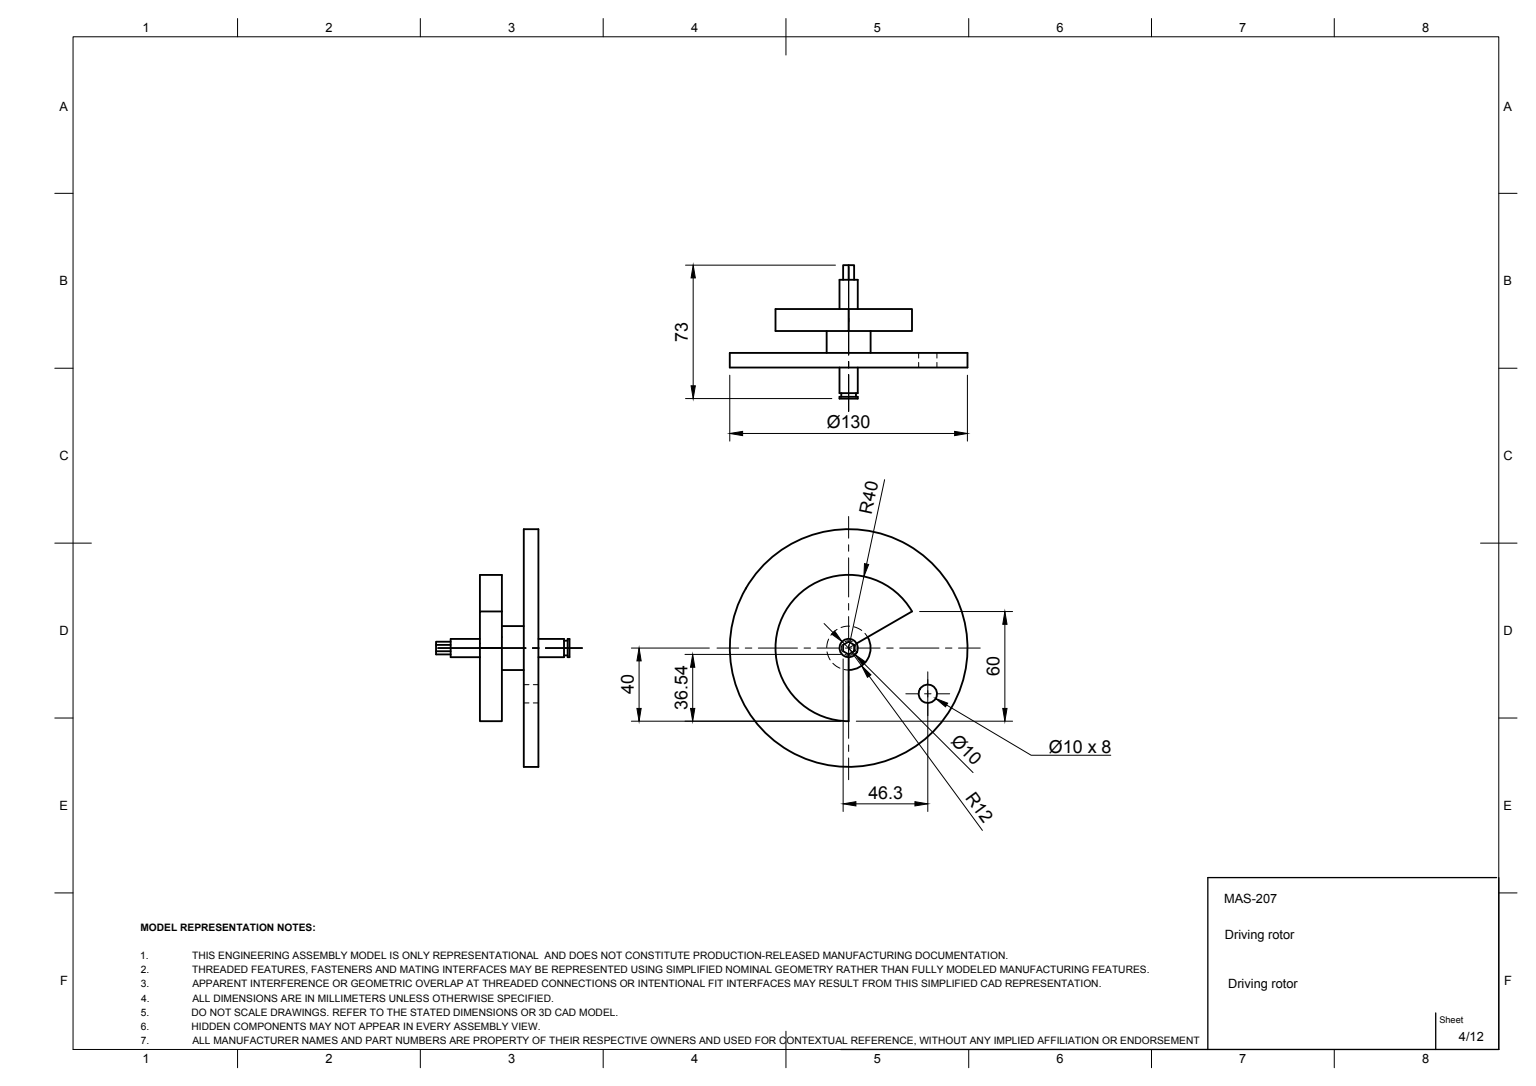
ISO-10303-21;
HEADER;
/* Generated by software containing ST-Developer
 * from STEP Tools, Inc. (www.steptools.com) 
 */

FILE_DESCRIPTION(
/* description */ ('Independent six-slot Geneva indexer. Center distance100, drive radius
50, 60degree indexing per input revolution with120degree engagement an
d240degree dwell. Native machined concave locking faces and relieved d
isk; replaceable retained drive pin; keyed output shaft. Geometry traj
ectory checks use calculated indexing positions, not a contact-dynamic
s simulation. No load or production rating assigned.'),
/* implementation_level */ '2;1');

FILE_NAME(
/* name */ 'Driving rotor.step',
/* time_stamp */ '2026-11-09T17:53:22-08:00',
/* author */ (''),
/* organization */ (''),
/* preprocessor_version */ 'ST-DEVELOPER v20.2',
/* originating_system */ 'Autodesk Translation Framework v15.17.0.0',
/* authorisation */ '');

FILE_SCHEMA (('AUTOMOTIVE_DESIGN { 1 0 10303 214 3 1 1 }'));
ENDSEC;

DATA;
#10=MECHANICAL_DESIGN_GEOMETRIC_PRESENTATION_REPRESENTATION('',(#102),#4149);
#80=SHAPE_REPRESENTATION_RELATIONSHIP('SRR','None',#4197,#91);
#91=ADVANCED_BREP_SHAPE_REPRESENTATION('',(#113),#4139);
#102=STYLED_ITEM('',(#4261),#113);
#113=MANIFOLD_SOLID_BREP('Body1',#2296);
#135=FACE_BOUND('',#407,.T.);
#136=FACE_BOUND('',#409,.T.);
#137=FACE_BOUND('',#421,.T.);
#138=FACE_BOUND('',#422,.T.);
#139=FACE_BOUND('',#424,.T.);
#140=FACE_BOUND('',#425,.T.);
#141=FACE_BOUND('',#430,.T.);
#167=PLANE('',#2455);
#168=PLANE('',#2456);
#169=PLANE('',#2457);
#170=PLANE('',#2458);
#171=PLANE('',#2459);
#172=PLANE('',#2460);
#173=PLANE('',#2461);
#174=PLANE('',#2465);
#175=PLANE('',#2467);
#176=PLANE('',#2474);
#177=PLANE('',#2476);
#178=PLANE('',#2478);
#179=PLANE('',#2479);
#180=PLANE('',#2480);
#181=PLANE('',#2484);
#182=PLANE('',#2491);
#183=PLANE('',#2493);
#184=PLANE('',#2500);
#185=PLANE('',#2501);
#250=FACE_OUTER_BOUND('',#398,.T.);
#251=FACE_OUTER_BOUND('',#399,.T.);
#252=FACE_OUTER_BOUND('',#400,.T.);
#253=FACE_OUTER_BOUND('',#401,.T.);
#254=FACE_OUTER_BOUND('',#402,.T.);
#255=FACE_OUTER_BOUND('',#403,.T.);
#256=FACE_OUTER_BOUND('',#404,.T.);
#257=FACE_OUTER_BOUND('',#405,.T.);
#258=FACE_OUTER_BOUND('',#406,.T.);
#259=FACE_OUTER_BOUND('',#408,.T.);
#260=FACE_OUTER_BOUND('',#410,.T.);
#261=FACE_OUTER_BOUND('',#411,.T.);
#262=FACE_OUTER_BOUND('',#412,.T.);
#263=FACE_OUTER_BOUND('',#413,.T.);
#264=FACE_OUTER_BOUND('',#414,.T.);
#265=FACE_OUTER_BOUND('',#415,.T.);
#266=FACE_OUTER_BOUND('',#416,.T.);
#267=FACE_OUTER_BOUND('',#417,.T.);
#268=FACE_OUTER_BOUND('',#418,.T.);
#269=FACE_OUTER_BOUND('',#419,.T.);
#270=FACE_OUTER_BOUND('',#420,.T.);
#271=FACE_OUTER_BOUND('',#423,.T.);
#272=FACE_OUTER_BOUND('',#426,.T.);
#273=FACE_OUTER_BOUND('',#427,.T.);
#274=FACE_OUTER_BOUND('',#428,.T.);
#275=FACE_OUTER_BOUND('',#429,.T.);
#276=FACE_OUTER_BOUND('',#431,.T.);
#398=EDGE_LOOP('',(#1568,#1569,#1570,#1571));
#399=EDGE_LOOP('',(#1572,#1573,#1574,#1575));
#400=EDGE_LOOP('',(#1576,#1577,#1578,#1579));
#401=EDGE_LOOP('',(#1580,#1581,#1582,#1583));
#402=EDGE_LOOP('',(#1584,#1585,#1586,#1587));
#403=EDGE_LOOP('',(#1588,#1589,#1590,#1591));
#404=EDGE_LOOP('',(#1592,#1593,#1594,#1595,#1596,#1597));
#405=EDGE_LOOP('',(#1598,#1599,#1600,#1601));
#406=EDGE_LOOP('',(#1602));
#407=EDGE_LOOP('',(#1603));
#408=EDGE_LOOP('',(#1604));
#409=EDGE_LOOP('',(#1605));
#410=EDGE_LOOP('',(#1606,#1607,#1608,#1609));
#411=EDGE_LOOP('',(#1610,#1611,#1612,#1613));
#412=EDGE_LOOP('',(#1614,#1615,#1616));
#413=EDGE_LOOP('',(#1617,#1618,#1619));
#414=EDGE_LOOP('',(#1620,#1621,#1622,#1623,#1624,#1625));
#415=EDGE_LOOP('',(#1626,#1627,#1628,#1629,#1630,#1631));
#416=EDGE_LOOP('',(#1632,#1633,#1634,#1635,#1636));
#417=EDGE_LOOP('',(#1637,#1638,#1639,#1640,#1641));
#418=EDGE_LOOP('',(#1642,#1643,#1644,#1645));
#419=EDGE_LOOP('',(#1646,#1647,#1648,#1649,#1650,#1651));
#420=EDGE_LOOP('',(#1652));
#421=EDGE_LOOP('',(#1653));
#422=EDGE_LOOP('',(#1654));
#423=EDGE_LOOP('',(#1655));
#424=EDGE_LOOP('',(#1656));
#425=EDGE_LOOP('',(#1657));
#426=EDGE_LOOP('',(#1658,#1659,#1660,#1661));
#427=EDGE_LOOP('',(#1662,#1663,#1664,#1665));
#428=EDGE_LOOP('',(#1666,#1667,#1668,#1669,#1670,#1671));
#429=EDGE_LOOP('',(#1672));
#430=EDGE_LOOP('',(#1673,#1674,#1675,#1676,#1677,#1678));
#431=EDGE_LOOP('',(#1679));
#566=LINE('',#3535,#738);
#567=LINE('',#3537,#739);
#568=LINE('',#3539,#740);
#569=LINE('',#3540,#741);
#570=LINE('',#3543,#742);
#571=LINE('',#3545,#743);
#572=LINE('',#3546,#744);
#573=LINE('',#3549,#745);
#574=LINE('',#3551,#746);
#575=LINE('',#3552,#747);
#576=LINE('',#3555,#748);
#577=LINE('',#3557,#749);
#578=LINE('',#3558,#750);
#579=LINE('',#3561,#751);
#580=LINE('',#3563,#752);
#581=LINE('',#3564,#753);
#582=LINE('',#3566,#754);
#583=LINE('',#3567,#755);
#584=LINE('',#3573,#756);
#585=LINE('',#3584,#757);
#586=LINE('',#3589,#758);
#587=LINE('',#3596,#759);
#588=LINE('',#3597,#760);
#589=LINE('',#3603,#761);
#590=LINE('',#3604,#762);
#591=LINE('',#3608,#763);
#592=LINE('',#3609,#764);
#593=LINE('',#3610,#765);
#594=LINE('',#3611,#766);
#595=LINE('',#3615,#767);
#596=LINE('',#3616,#768);
#597=LINE('',#3617,#769);
#598=LINE('',#3631,#770);
#599=LINE('',#3640,#771);
#600=LINE('',#3643,#772);
#601=LINE('',#3648,#773);
#738=VECTOR('',#2791,10.);
#739=VECTOR('',#2792,10.);
#740=VECTOR('',#2793,10.);
#741=VECTOR('',#2794,10.);
#742=VECTOR('',#2797,10.);
#743=VECTOR('',#2798,10.);
#744=VECTOR('',#2799,10.);
#745=VECTOR('',#2802,10.);
#746=VECTOR('',#2803,10.);
#747=VECTOR('',#2804,10.);
#748=VECTOR('',#2807,10.);
#749=VECTOR('',#2808,10.);
#750=VECTOR('',#2809,10.);
#751=VECTOR('',#2812,10.);
#752=VECTOR('',#2813,10.);
#753=VECTOR('',#2814,10.);
#754=VECTOR('',#2817,10.);
#755=VECTOR('',#2818,10.);
#756=VECTOR('',#2825,4.);
#757=VECTOR('',#2840,5.);
#758=VECTOR('',#2845,5.);
#759=VECTOR('',#2852,10.);
#760=VECTOR('',#2853,10.);
#761=VECTOR('',#2858,10.);
#762=VECTOR('',#2859,10.);
#763=VECTOR('',#2862,10.);
#764=VECTOR('',#2863,10.);
#765=VECTOR('',#2864,10.);
#766=VECTOR('',#2865,10.);
#767=VECTOR('',#2868,10.);
#768=VECTOR('',#2869,10.);
#769=VECTOR('',#2870,10.);
#770=VECTOR('',#2891,12.);
#771=VECTOR('',#2904,60.);
#772=VECTOR('',#2907,5.);
#773=VECTOR('',#2914,5.);
#904=CIRCLE('',#2463,4.);
#905=CIRCLE('',#2464,4.);
#906=CIRCLE('',#2466,5.);
#907=CIRCLE('',#2468,5.);
#908=CIRCLE('',#2470,5.);
#909=CIRCLE('',#2472,5.);
#910=CIRCLE('',#2473,5.);
#911=CIRCLE('',#2475,5.);
#912=CIRCLE('',#2477,12.);
#913=CIRCLE('',#2481,5.);
#914=CIRCLE('',#2482,5.);
#915=CIRCLE('',#2483,40.);
#916=CIRCLE('',#2485,40.);
#917=CIRCLE('',#2486,12.);
#918=CIRCLE('',#2487,12.);
#919=CIRCLE('',#2490,12.);
#920=CIRCLE('',#2492,65.);
#921=CIRCLE('',#2494,65.);
#922=CIRCLE('',#2497,5.);
#923=CIRCLE('',#2499,5.);
#1036=VERTEX_POINT('',#3533);
#1037=VERTEX_POINT('',#3534);
#1038=VERTEX_POINT('',#3536);
#1039=VERTEX_POINT('',#3538);
#1040=VERTEX_POINT('',#3542);
#1041=VERTEX_POINT('',#3544);
#1042=VERTEX_POINT('',#3548);
#1043=VERTEX_POINT('',#3550);
#1044=VERTEX_POINT('',#3554);
#1045=VERTEX_POINT('',#3556);
#1046=VERTEX_POINT('',#3560);
#1047=VERTEX_POINT('',#3562);
#1048=VERTEX_POINT('',#3570);
#1049=VERTEX_POINT('',#3572);
#1050=VERTEX_POINT('',#3576);
#1051=VERTEX_POINT('',#3579);
#1052=VERTEX_POINT('',#3582);
#1053=VERTEX_POINT('',#3586);
#1054=VERTEX_POINT('',#3588);
#1055=VERTEX_POINT('',#3592);
#1056=VERTEX_POINT('',#3593);
#1057=VERTEX_POINT('',#3595);
#1058=VERTEX_POINT('',#3599);
#1059=VERTEX_POINT('',#3600);
#1060=VERTEX_POINT('',#3602);
#1061=VERTEX_POINT('',#3606);
#1062=VERTEX_POINT('',#3607);
#1063=VERTEX_POINT('',#3613);
#1064=VERTEX_POINT('',#3614);
#1065=VERTEX_POINT('',#3619);
#1066=VERTEX_POINT('',#3625);
#1067=VERTEX_POINT('',#3630);
#1068=VERTEX_POINT('',#3634);
#1069=VERTEX_POINT('',#3637);
#1070=VERTEX_POINT('',#3642);
#1071=VERTEX_POINT('',#3646);
#1242=EDGE_CURVE('',#1036,#1037,#566,.T.);
#1243=EDGE_CURVE('',#1036,#1038,#567,.T.);
#1244=EDGE_CURVE('',#1039,#1038,#568,.T.);
#1245=EDGE_CURVE('',#1037,#1039,#569,.T.);
#1246=EDGE_CURVE('',#1037,#1040,#570,.T.);
#1247=EDGE_CURVE('',#1041,#1039,#571,.T.);
#1248=EDGE_CURVE('',#1040,#1041,#572,.T.);
#1249=EDGE_CURVE('',#1040,#1042,#573,.T.);
#1250=EDGE_CURVE('',#1043,#1041,#574,.T.);
#1251=EDGE_CURVE('',#1042,#1043,#575,.T.);
#1252=EDGE_CURVE('',#1042,#1044,#576,.T.);
#1253=EDGE_CURVE('',#1045,#1043,#577,.T.);
#1254=EDGE_CURVE('',#1044,#1045,#578,.T.);
#1255=EDGE_CURVE('',#1044,#1046,#579,.T.);
#1256=EDGE_CURVE('',#1047,#1045,#580,.T.);
#1257=EDGE_CURVE('',#1046,#1047,#581,.T.);
#1258=EDGE_CURVE('',#1046,#1036,#582,.T.);
#1259=EDGE_CURVE('',#1038,#1047,#583,.T.);
#1260=EDGE_CURVE('',#1048,#1048,#904,.T.);
#1261=EDGE_CURVE('',#1048,#1049,#584,.T.);
#1262=EDGE_CURVE('',#1049,#1049,#905,.T.);
#1263=EDGE_CURVE('',#1050,#1050,#906,.T.);
#1264=EDGE_CURVE('',#1051,#1051,#907,.T.);
#1265=EDGE_CURVE('',#1052,#1052,#908,.T.);
#1266=EDGE_CURVE('',#1052,#1051,#585,.T.);
#1267=EDGE_CURVE('',#1053,#1053,#909,.T.);
#1268=EDGE_CURVE('',#1053,#1054,#586,.T.);
#1269=EDGE_CURVE('',#1054,#1054,#910,.T.);
#1270=EDGE_CURVE('',#1055,#1056,#911,.T.);
#1271=EDGE_CURVE('',#1057,#1055,#587,.T.);
#1272=EDGE_CURVE('',#1056,#1057,#588,.T.);
#1273=EDGE_CURVE('',#1058,#1059,#912,.T.);
#1274=EDGE_CURVE('',#1060,#1059,#589,.T.);
#1275=EDGE_CURVE('',#1058,#1060,#590,.T.);
#1276=EDGE_CURVE('',#1061,#1062,#591,.T.);
#1277=EDGE_CURVE('',#1056,#1061,#592,.T.);
#1278=EDGE_CURVE('',#1057,#1060,#593,.T.);
#1279=EDGE_CURVE('',#1062,#1059,#594,.T.);
#1280=EDGE_CURVE('',#1063,#1064,#595,.T.);
#1281=EDGE_CURVE('',#1058,#1063,#596,.T.);
#1282=EDGE_CURVE('',#1064,#1055,#597,.T.);
#1283=EDGE_CURVE('',#1065,#1055,#913,.T.);
#1284=EDGE_CURVE('',#1056,#1065,#914,.T.);
#1285=EDGE_CURVE('',#1061,#1064,#915,.T.);
#1286=EDGE_CURVE('',#1062,#1063,#916,.T.);
#1287=EDGE_CURVE('',#1059,#1066,#917,.T.);
#1288=EDGE_CURVE('',#1066,#1058,#918,.T.);
#1289=EDGE_CURVE('',#1066,#1067,#598,.T.);
#1290=EDGE_CURVE('',#1067,#1067,#919,.T.);
#1291=EDGE_CURVE('',#1068,#1068,#920,.F.);
#1292=EDGE_CURVE('',#1069,#1069,#921,.F.);
#1293=EDGE_CURVE('',#1068,#1069,#599,.T.);
#1294=EDGE_CURVE('',#1050,#1070,#600,.T.);
#1295=EDGE_CURVE('',#1070,#1070,#922,.T.);
#1296=EDGE_CURVE('',#1071,#1071,#923,.T.);
#1297=EDGE_CURVE('',#1071,#1065,#601,.T.);
#1568=ORIENTED_EDGE('',*,*,#1242,.F.);
#1569=ORIENTED_EDGE('',*,*,#1243,.T.);
#1570=ORIENTED_EDGE('',*,*,#1244,.F.);
#1571=ORIENTED_EDGE('',*,*,#1245,.F.);
#1572=ORIENTED_EDGE('',*,*,#1246,.F.);
#1573=ORIENTED_EDGE('',*,*,#1245,.T.);
#1574=ORIENTED_EDGE('',*,*,#1247,.F.);
#1575=ORIENTED_EDGE('',*,*,#1248,.F.);
#1576=ORIENTED_EDGE('',*,*,#1249,.F.);
#1577=ORIENTED_EDGE('',*,*,#1248,.T.);
#1578=ORIENTED_EDGE('',*,*,#1250,.F.);
#1579=ORIENTED_EDGE('',*,*,#1251,.F.);
#1580=ORIENTED_EDGE('',*,*,#1252,.F.);
#1581=ORIENTED_EDGE('',*,*,#1251,.T.);
#1582=ORIENTED_EDGE('',*,*,#1253,.F.);
#1583=ORIENTED_EDGE('',*,*,#1254,.F.);
#1584=ORIENTED_EDGE('',*,*,#1255,.F.);
#1585=ORIENTED_EDGE('',*,*,#1254,.T.);
#1586=ORIENTED_EDGE('',*,*,#1256,.F.);
#1587=ORIENTED_EDGE('',*,*,#1257,.F.);
#1588=ORIENTED_EDGE('',*,*,#1258,.F.);
#1589=ORIENTED_EDGE('',*,*,#1257,.T.);
#1590=ORIENTED_EDGE('',*,*,#1259,.F.);
#1591=ORIENTED_EDGE('',*,*,#1243,.F.);
#1592=ORIENTED_EDGE('',*,*,#1259,.T.);
#1593=ORIENTED_EDGE('',*,*,#1256,.T.);
#1594=ORIENTED_EDGE('',*,*,#1253,.T.);
#1595=ORIENTED_EDGE('',*,*,#1250,.T.);
#1596=ORIENTED_EDGE('',*,*,#1247,.T.);
#1597=ORIENTED_EDGE('',*,*,#1244,.T.);
#1598=ORIENTED_EDGE('',*,*,#1260,.T.);
#1599=ORIENTED_EDGE('',*,*,#1261,.T.);
#1600=ORIENTED_EDGE('',*,*,#1262,.F.);
#1601=ORIENTED_EDGE('',*,*,#1261,.F.);
#1602=ORIENTED_EDGE('',*,*,#1263,.F.);
#1603=ORIENTED_EDGE('',*,*,#1260,.F.);
#1604=ORIENTED_EDGE('',*,*,#1264,.F.);
#1605=ORIENTED_EDGE('',*,*,#1262,.T.);
#1606=ORIENTED_EDGE('',*,*,#1265,.T.);
#1607=ORIENTED_EDGE('',*,*,#1266,.T.);
#1608=ORIENTED_EDGE('',*,*,#1264,.T.);
#1609=ORIENTED_EDGE('',*,*,#1266,.F.);
#1610=ORIENTED_EDGE('',*,*,#1267,.F.);
#1611=ORIENTED_EDGE('',*,*,#1268,.T.);
#1612=ORIENTED_EDGE('',*,*,#1269,.F.);
#1613=ORIENTED_EDGE('',*,*,#1268,.F.);
#1614=ORIENTED_EDGE('',*,*,#1270,.F.);
#1615=ORIENTED_EDGE('',*,*,#1271,.F.);
#1616=ORIENTED_EDGE('',*,*,#1272,.F.);
#1617=ORIENTED_EDGE('',*,*,#1273,.T.);
#1618=ORIENTED_EDGE('',*,*,#1274,.F.);
#1619=ORIENTED_EDGE('',*,*,#1275,.F.);
#1620=ORIENTED_EDGE('',*,*,#1276,.F.);
#1621=ORIENTED_EDGE('',*,*,#1277,.F.);
#1622=ORIENTED_EDGE('',*,*,#1272,.T.);
#1623=ORIENTED_EDGE('',*,*,#1278,.T.);
#1624=ORIENTED_EDGE('',*,*,#1274,.T.);
#1625=ORIENTED_EDGE('',*,*,#1279,.F.);
#1626=ORIENTED_EDGE('',*,*,#1280,.F.);
#1627=ORIENTED_EDGE('',*,*,#1281,.F.);
#1628=ORIENTED_EDGE('',*,*,#1275,.T.);
#1629=ORIENTED_EDGE('',*,*,#1278,.F.);
#1630=ORIENTED_EDGE('',*,*,#1271,.T.);
#1631=ORIENTED_EDGE('',*,*,#1282,.F.);
#1632=ORIENTED_EDGE('',*,*,#1282,.T.);
#1633=ORIENTED_EDGE('',*,*,#1283,.F.);
#1634=ORIENTED_EDGE('',*,*,#1284,.F.);
#1635=ORIENTED_EDGE('',*,*,#1277,.T.);
#1636=ORIENTED_EDGE('',*,*,#1285,.T.);
#1637=ORIENTED_EDGE('',*,*,#1281,.T.);
#1638=ORIENTED_EDGE('',*,*,#1286,.F.);
#1639=ORIENTED_EDGE('',*,*,#1279,.T.);
#1640=ORIENTED_EDGE('',*,*,#1287,.T.);
#1641=ORIENTED_EDGE('',*,*,#1288,.T.);
#1642=ORIENTED_EDGE('',*,*,#1280,.T.);
#1643=ORIENTED_EDGE('',*,*,#1285,.F.);
#1644=ORIENTED_EDGE('',*,*,#1276,.T.);
#1645=ORIENTED_EDGE('',*,*,#1286,.T.);
#1646=ORIENTED_EDGE('',*,*,#1287,.F.);
#1647=ORIENTED_EDGE('',*,*,#1273,.F.);
#1648=ORIENTED_EDGE('',*,*,#1288,.F.);
#1649=ORIENTED_EDGE('',*,*,#1289,.T.);
#1650=ORIENTED_EDGE('',*,*,#1290,.F.);
#1651=ORIENTED_EDGE('',*,*,#1289,.F.);
#1652=ORIENTED_EDGE('',*,*,#1291,.T.);
#1653=ORIENTED_EDGE('',*,*,#1267,.T.);
#1654=ORIENTED_EDGE('',*,*,#1290,.T.);
#1655=ORIENTED_EDGE('',*,*,#1292,.F.);
#1656=ORIENTED_EDGE('',*,*,#1269,.T.);
#1657=ORIENTED_EDGE('',*,*,#1265,.F.);
#1658=ORIENTED_EDGE('',*,*,#1291,.F.);
#1659=ORIENTED_EDGE('',*,*,#1293,.T.);
#1660=ORIENTED_EDGE('',*,*,#1292,.T.);
#1661=ORIENTED_EDGE('',*,*,#1293,.F.);
#1662=ORIENTED_EDGE('',*,*,#1263,.T.);
#1663=ORIENTED_EDGE('',*,*,#1294,.T.);
#1664=ORIENTED_EDGE('',*,*,#1295,.T.);
#1665=ORIENTED_EDGE('',*,*,#1294,.F.);
#1666=ORIENTED_EDGE('',*,*,#1296,.F.);
#1667=ORIENTED_EDGE('',*,*,#1297,.T.);
#1668=ORIENTED_EDGE('',*,*,#1283,.T.);
#1669=ORIENTED_EDGE('',*,*,#1270,.T.);
#1670=ORIENTED_EDGE('',*,*,#1284,.T.);
#1671=ORIENTED_EDGE('',*,*,#1297,.F.);
#1672=ORIENTED_EDGE('',*,*,#1296,.T.);
#1673=ORIENTED_EDGE('',*,*,#1242,.T.);
#1674=ORIENTED_EDGE('',*,*,#1246,.T.);
#1675=ORIENTED_EDGE('',*,*,#1249,.T.);
#1676=ORIENTED_EDGE('',*,*,#1252,.T.);
#1677=ORIENTED_EDGE('',*,*,#1255,.T.);
#1678=ORIENTED_EDGE('',*,*,#1258,.T.);
#1679=ORIENTED_EDGE('',*,*,#1295,.F.);
#2106=CYLINDRICAL_SURFACE('',#2462,4.);
#2107=CYLINDRICAL_SURFACE('',#2469,5.);
#2108=CYLINDRICAL_SURFACE('',#2471,5.);
#2109=CYLINDRICAL_SURFACE('',#2488,40.);
#2110=CYLINDRICAL_SURFACE('',#2489,12.);
#2111=CYLINDRICAL_SURFACE('',#2495,65.);
#2112=CYLINDRICAL_SURFACE('',#2496,5.);
#2113=CYLINDRICAL_SURFACE('',#2498,5.);
#2171=ADVANCED_FACE('',(#250),#167,.T.);
#2172=ADVANCED_FACE('',(#251),#168,.T.);
#2173=ADVANCED_FACE('',(#252),#169,.T.);
#2174=ADVANCED_FACE('',(#253),#170,.T.);
#2175=ADVANCED_FACE('',(#254),#171,.T.);
#2176=ADVANCED_FACE('',(#255),#172,.T.);
#2177=ADVANCED_FACE('',(#256),#173,.T.);
#2178=ADVANCED_FACE('',(#257),#2106,.T.);
#2179=ADVANCED_FACE('',(#258,#135),#174,.F.);
#2180=ADVANCED_FACE('',(#259,#136),#175,.F.);
#2181=ADVANCED_FACE('',(#260),#2107,.T.);
#2182=ADVANCED_FACE('',(#261),#2108,.F.);
#2183=ADVANCED_FACE('',(#262),#176,.F.);
#2184=ADVANCED_FACE('',(#263),#177,.F.);
#2185=ADVANCED_FACE('',(#264),#178,.F.);
#2186=ADVANCED_FACE('',(#265),#179,.F.);
#2187=ADVANCED_FACE('',(#266),#180,.T.);
#2188=ADVANCED_FACE('',(#267),#181,.F.);
#2189=ADVANCED_FACE('',(#268),#2109,.T.);
#2190=ADVANCED_FACE('',(#269),#2110,.T.);
#2191=ADVANCED_FACE('',(#270,#137,#138),#182,.T.);
#2192=ADVANCED_FACE('',(#271,#139,#140),#183,.F.);
#2193=ADVANCED_FACE('',(#272),#2111,.T.);
#2194=ADVANCED_FACE('',(#273),#2112,.T.);
#2195=ADVANCED_FACE('',(#274),#2113,.T.);
#2196=ADVANCED_FACE('',(#275,#141),#184,.T.);
#2197=ADVANCED_FACE('',(#276),#185,.F.);
#2296=CLOSED_SHELL('',(#2171,#2172,#2173,#2174,#2175,#2176,#2177,#2178,
#2179,#2180,#2181,#2182,#2183,#2184,#2185,#2186,#2187,#2188,#2189,#2190,
#2191,#2192,#2193,#2194,#2195,#2196,#2197));
#2454=AXIS2_PLACEMENT_3D('',#3531,#2787,#2788);
#2455=AXIS2_PLACEMENT_3D('',#3532,#2789,#2790);
#2456=AXIS2_PLACEMENT_3D('',#3541,#2795,#2796);
#2457=AXIS2_PLACEMENT_3D('',#3547,#2800,#2801);
#2458=AXIS2_PLACEMENT_3D('',#3553,#2805,#2806);
#2459=AXIS2_PLACEMENT_3D('',#3559,#2810,#2811);
#2460=AXIS2_PLACEMENT_3D('',#3565,#2815,#2816);
#2461=AXIS2_PLACEMENT_3D('',#3568,#2819,#2820);
#2462=AXIS2_PLACEMENT_3D('',#3569,#2821,#2822);
#2463=AXIS2_PLACEMENT_3D('',#3571,#2823,#2824);
#2464=AXIS2_PLACEMENT_3D('',#3574,#2826,#2827);
#2465=AXIS2_PLACEMENT_3D('',#3575,#2828,#2829);
#2466=AXIS2_PLACEMENT_3D('',#3577,#2830,#2831);
#2467=AXIS2_PLACEMENT_3D('',#3578,#2832,#2833);
#2468=AXIS2_PLACEMENT_3D('',#3580,#2834,#2835);
#2469=AXIS2_PLACEMENT_3D('',#3581,#2836,#2837);
#2470=AXIS2_PLACEMENT_3D('',#3583,#2838,#2839);
#2471=AXIS2_PLACEMENT_3D('',#3585,#2841,#2842);
#2472=AXIS2_PLACEMENT_3D('',#3587,#2843,#2844);
#2473=AXIS2_PLACEMENT_3D('',#3590,#2846,#2847);
#2474=AXIS2_PLACEMENT_3D('',#3591,#2848,#2849);
#2475=AXIS2_PLACEMENT_3D('',#3594,#2850,#2851);
#2476=AXIS2_PLACEMENT_3D('',#3598,#2854,#2855);
#2477=AXIS2_PLACEMENT_3D('',#3601,#2856,#2857);
#2478=AXIS2_PLACEMENT_3D('',#3605,#2860,#2861);
#2479=AXIS2_PLACEMENT_3D('',#3612,#2866,#2867);
#2480=AXIS2_PLACEMENT_3D('',#3618,#2871,#2872);
#2481=AXIS2_PLACEMENT_3D('',#3620,#2873,#2874);
#2482=AXIS2_PLACEMENT_3D('',#3621,#2875,#2876);
#2483=AXIS2_PLACEMENT_3D('',#3622,#2877,#2878);
#2484=AXIS2_PLACEMENT_3D('',#3623,#2879,#2880);
#2485=AXIS2_PLACEMENT_3D('',#3624,#2881,#2882);
#2486=AXIS2_PLACEMENT_3D('',#3626,#2883,#2884);
#2487=AXIS2_PLACEMENT_3D('',#3627,#2885,#2886);
#2488=AXIS2_PLACEMENT_3D('',#3628,#2887,#2888);
#2489=AXIS2_PLACEMENT_3D('',#3629,#2889,#2890);
#2490=AXIS2_PLACEMENT_3D('',#3632,#2892,#2893);
#2491=AXIS2_PLACEMENT_3D('',#3633,#2894,#2895);
#2492=AXIS2_PLACEMENT_3D('',#3635,#2896,#2897);
#2493=AXIS2_PLACEMENT_3D('',#3636,#2898,#2899);
#2494=AXIS2_PLACEMENT_3D('',#3638,#2900,#2901);
#2495=AXIS2_PLACEMENT_3D('',#3639,#2902,#2903);
#2496=AXIS2_PLACEMENT_3D('',#3641,#2905,#2906);
#2497=AXIS2_PLACEMENT_3D('',#3644,#2908,#2909);
#2498=AXIS2_PLACEMENT_3D('',#3645,#2910,#2911);
#2499=AXIS2_PLACEMENT_3D('',#3647,#2912,#2913);
#2500=AXIS2_PLACEMENT_3D('',#3649,#2915,#2916);
#2501=AXIS2_PLACEMENT_3D('',#3650,#2917,#2918);
#2787=DIRECTION('axis',(0.,0.,1.));
#2788=DIRECTION('refdir',(1.,0.,0.));
#2789=DIRECTION('center_axis',(-1.60246890531964E-16,-1.,0.));
#2790=DIRECTION('ref_axis',(1.,-1.60246890531964E-16,0.));
#2791=DIRECTION('',(-1.,1.60246890531964E-16,0.));
#2792=DIRECTION('',(0.,0.,1.));
#2793=DIRECTION('',(1.,-1.60246890531964E-16,0.));
#2794=DIRECTION('',(0.,0.,1.));
#2795=DIRECTION('center_axis',(-0.866025403784439,-0.5,0.));
#2796=DIRECTION('ref_axis',(0.5,-0.866025403784439,0.));
#2797=DIRECTION('',(-0.5,0.866025403784439,0.));
#2798=DIRECTION('',(0.5,-0.866025403784439,0.));
#2799=DIRECTION('',(0.,0.,1.));
#2800=DIRECTION('center_axis',(-0.866025403784439,0.5,0.));
#2801=DIRECTION('ref_axis',(-0.5,-0.866025403784439,0.));
#2802=DIRECTION('',(0.5,0.866025403784439,0.));
#2803=DIRECTION('',(-0.5,-0.866025403784439,0.));
#2804=DIRECTION('',(0.,0.,1.));
#2805=DIRECTION('center_axis',(1.60246890531964E-16,1.,0.));
#2806=DIRECTION('ref_axis',(-1.,1.60246890531964E-16,0.));
#2807=DIRECTION('',(1.,-1.60246890531964E-16,0.));
#2808=DIRECTION('',(-1.,1.60246890531964E-16,0.));
#2809=DIRECTION('',(0.,0.,1.));
#2810=DIRECTION('center_axis',(0.866025403784439,0.5,0.));
#2811=DIRECTION('ref_axis',(-0.5,0.866025403784439,0.));
#2812=DIRECTION('',(0.5,-0.866025403784439,0.));
#2813=DIRECTION('',(-0.5,0.866025403784439,0.));
#2814=DIRECTION('',(0.,0.,1.));
#2815=DIRECTION('center_axis',(0.866025403784439,-0.5,0.));
#2816=DIRECTION('ref_axis',(0.5,0.866025403784439,0.));
#2817=DIRECTION('',(-0.5,-0.866025403784439,0.));
#2818=DIRECTION('',(0.5,0.866025403784439,0.));
#2819=DIRECTION('center_axis',(0.,0.,1.));
#2820=DIRECTION('ref_axis',(1.,0.,0.));
#2821=DIRECTION('center_axis',(0.,0.,1.));
#2822=DIRECTION('ref_axis',(1.,0.,0.));
#2823=DIRECTION('center_axis',(0.,0.,1.));
#2824=DIRECTION('ref_axis',(1.,0.,0.));
#2825=DIRECTION('',(0.,0.,1.));
#2826=DIRECTION('center_axis',(0.,0.,1.));
#2827=DIRECTION('ref_axis',(1.,0.,0.));
#2828=DIRECTION('center_axis',(0.,0.,-1.));
#2829=DIRECTION('ref_axis',(-1.,0.,0.));
#2830=DIRECTION('center_axis',(0.,0.,-1.));
#2831=DIRECTION('ref_axis',(1.,0.,0.));
#2832=DIRECTION('center_axis',(0.,0.,1.));
#2833=DIRECTION('ref_axis',(1.,0.,0.));
#2834=DIRECTION('center_axis',(0.,0.,1.));
#2835=DIRECTION('ref_axis',(1.,0.,0.));
#2836=DIRECTION('center_axis',(0.,0.,1.));
#2837=DIRECTION('ref_axis',(1.,0.,0.));
#2838=DIRECTION('center_axis',(0.,0.,-1.));
#2839=DIRECTION('ref_axis',(1.,0.,0.));
#2840=DIRECTION('',(0.,0.,-1.));
#2841=DIRECTION('center_axis',(0.,0.,-1.));
#2842=DIRECTION('ref_axis',(1.,0.,0.));
#2843=DIRECTION('center_axis',(0.,0.,-1.));
#2844=DIRECTION('ref_axis',(1.,0.,0.));
#2845=DIRECTION('',(0.,0.,-1.));
#2846=DIRECTION('center_axis',(0.,0.,1.));
#2847=DIRECTION('ref_axis',(1.,0.,0.));
#2848=DIRECTION('center_axis',(0.,0.,1.));
#2849=DIRECTION('ref_axis',(1.,0.,0.));
#2850=DIRECTION('center_axis',(0.,0.,1.));
#2851=DIRECTION('ref_axis',(1.,0.,0.));
#2852=DIRECTION('',(0.5,-0.866025403784439,0.));
#2853=DIRECTION('',(-0.5,-0.866025403784439,0.));
#2854=DIRECTION('center_axis',(0.,0.,-1.));
#2855=DIRECTION('ref_axis',(-1.,0.,0.));
#2856=DIRECTION('center_axis',(0.,0.,1.));
#2857=DIRECTION('ref_axis',(1.,0.,0.));
#2858=DIRECTION('',(0.5,0.866025403784439,0.));
#2859=DIRECTION('',(-0.5,0.866025403784439,0.));
#2860=DIRECTION('center_axis',(-0.866025403784439,0.5,0.));
#2861=DIRECTION('ref_axis',(0.5,0.866025403784439,0.));
#2862=DIRECTION('',(0.,0.,-1.));
#2863=DIRECTION('',(0.5,0.866025403784439,0.));
#2864=DIRECTION('',(0.,0.,-1.));
#2865=DIRECTION('',(-0.5,-0.866025403784439,0.));
#2866=DIRECTION('center_axis',(-0.866025403784439,-0.5,0.));
#2867=DIRECTION('ref_axis',(-0.5,0.866025403784439,0.));
#2868=DIRECTION('',(0.,0.,1.));
#2869=DIRECTION('',(0.5,-0.866025403784439,0.));
#2870=DIRECTION('',(-0.5,0.866025403784439,0.));
#2871=DIRECTION('center_axis',(0.,0.,1.));
#2872=DIRECTION('ref_axis',(1.,0.,0.));
#2873=DIRECTION('center_axis',(0.,0.,1.));
#2874=DIRECTION('ref_axis',(1.,0.,0.));
#2875=DIRECTION('center_axis',(0.,0.,1.));
#2876=DIRECTION('ref_axis',(1.,0.,0.));
#2877=DIRECTION('center_axis',(0.,0.,1.));
#2878=DIRECTION('ref_axis',(1.,0.,0.));
#2879=DIRECTION('center_axis',(0.,0.,1.));
#2880=DIRECTION('ref_axis',(1.,0.,0.));
#2881=DIRECTION('center_axis',(0.,0.,1.));
#2882=DIRECTION('ref_axis',(1.,0.,0.));
#2883=DIRECTION('center_axis',(0.,0.,1.));
#2884=DIRECTION('ref_axis',(1.,0.,0.));
#2885=DIRECTION('center_axis',(0.,0.,1.));
#2886=DIRECTION('ref_axis',(1.,0.,0.));
#2887=DIRECTION('center_axis',(0.,0.,1.));
#2888=DIRECTION('ref_axis',(-1.,-1.22464679914735E-16,0.));
#2889=DIRECTION('center_axis',(0.,0.,1.));
#2890=DIRECTION('ref_axis',(1.,0.,0.));
#2891=DIRECTION('',(0.,0.,-1.));
#2892=DIRECTION('center_axis',(0.,0.,-1.));
#2893=DIRECTION('ref_axis',(1.,0.,0.));
#2894=DIRECTION('center_axis',(0.,0.,1.));
#2895=DIRECTION('ref_axis',(1.,0.,0.));
#2896=DIRECTION('center_axis',(0.,0.,-1.));
#2897=DIRECTION('ref_axis',(1.,0.,0.));
#2898=DIRECTION('center_axis',(0.,0.,1.));
#2899=DIRECTION('ref_axis',(1.,0.,0.));
#2900=DIRECTION('center_axis',(0.,0.,-1.));
#2901=DIRECTION('ref_axis',(1.,0.,0.));
#2902=DIRECTION('center_axis',(0.,0.,1.));
#2903=DIRECTION('ref_axis',(1.,0.,0.));
#2904=DIRECTION('',(0.,0.,-1.));
#2905=DIRECTION('center_axis',(0.,0.,1.));
#2906=DIRECTION('ref_axis',(1.,0.,0.));
#2907=DIRECTION('',(0.,0.,-1.));
#2908=DIRECTION('center_axis',(0.,0.,1.));
#2909=DIRECTION('ref_axis',(1.,0.,0.));
#2910=DIRECTION('center_axis',(0.,0.,1.));
#2911=DIRECTION('ref_axis',(1.,0.,0.));
#2912=DIRECTION('center_axis',(0.,0.,1.));
#2913=DIRECTION('ref_axis',(1.,0.,0.));
#2914=DIRECTION('',(0.,0.,-1.));
#2915=DIRECTION('center_axis',(0.,0.,1.));
#2916=DIRECTION('ref_axis',(1.,0.,0.));
#2917=DIRECTION('center_axis',(0.,0.,1.));
#2918=DIRECTION('ref_axis',(1.,0.,0.));
#3531=CARTESIAN_POINT('',(0.,0.,0.));
#3532=CARTESIAN_POINT('Origin',(-1.73205080756888,-3.,60.));
#3533=CARTESIAN_POINT('',(1.73205080756888,-3.,60.));
#3534=CARTESIAN_POINT('',(-1.73205080756888,-3.,60.));
#3535=CARTESIAN_POINT('',(-0.86602540378444,-3.,60.));
#3536=CARTESIAN_POINT('',(1.73205080756888,-3.,68.));
#3537=CARTESIAN_POINT('',(1.73205080756888,-3.,60.));
#3538=CARTESIAN_POINT('',(-1.73205080756888,-3.,68.));
#3539=CARTESIAN_POINT('',(-1.73205080756888,-3.,68.));
#3540=CARTESIAN_POINT('',(-1.73205080756888,-3.,60.));
#3541=CARTESIAN_POINT('Origin',(-3.46410161513775,4.24230095489963E-16,
60.));
#3542=CARTESIAN_POINT('',(-3.46410161513775,4.24230095489963E-16,60.));
#3543=CARTESIAN_POINT('',(-3.03108891324554,-0.749999999999999,60.));
#3544=CARTESIAN_POINT('',(-3.46410161513775,5.55111512312578E-16,68.));
#3545=CARTESIAN_POINT('',(-3.46410161513775,4.24230095489963E-16,68.));
#3546=CARTESIAN_POINT('',(-3.46410161513775,4.24230095489963E-16,60.));
#3547=CARTESIAN_POINT('Origin',(-1.73205080756888,3.,60.));
#3548=CARTESIAN_POINT('',(-1.73205080756888,3.,60.));
#3549=CARTESIAN_POINT('',(-2.1650635094611,2.25,60.));
#3550=CARTESIAN_POINT('',(-1.73205080756888,3.,68.));
#3551=CARTESIAN_POINT('',(-1.73205080756888,3.,68.));
#3552=CARTESIAN_POINT('',(-1.73205080756888,3.,60.));
#3553=CARTESIAN_POINT('Origin',(1.73205080756888,3.,60.));
#3554=CARTESIAN_POINT('',(1.73205080756888,3.,60.));
#3555=CARTESIAN_POINT('',(0.866025403784439,3.,60.));
#3556=CARTESIAN_POINT('',(1.73205080756888,3.,68.));
#3557=CARTESIAN_POINT('',(1.73205080756888,3.,68.));
#3558=CARTESIAN_POINT('',(1.73205080756888,3.,60.));
#3559=CARTESIAN_POINT('Origin',(3.46410161513775,0.,60.));
#3560=CARTESIAN_POINT('',(3.46410161513775,0.,60.));
#3561=CARTESIAN_POINT('',(3.03108891324554,0.75,60.));
#3562=CARTESIAN_POINT('',(3.46410161513775,0.,68.));
#3563=CARTESIAN_POINT('',(3.46410161513775,0.,68.));
#3564=CARTESIAN_POINT('',(3.46410161513775,0.,60.));
#3565=CARTESIAN_POINT('Origin',(1.73205080756888,-3.,60.));
#3566=CARTESIAN_POINT('',(2.1650635094611,-2.25,60.));
#3567=CARTESIAN_POINT('',(1.73205080756888,-3.,68.));
#3568=CARTESIAN_POINT('Origin',(0.,5.55111512312578E-16,68.));
#3569=CARTESIAN_POINT('Origin',(0.,0.,-3.));
#3570=CARTESIAN_POINT('',(-4.,-4.89858719658941E-16,-4.));
#3571=CARTESIAN_POINT('Origin',(0.,0.,-4.));
#3572=CARTESIAN_POINT('',(-4.,-4.89858719658941E-16,-2.));
#3573=CARTESIAN_POINT('',(-4.,-4.89858719658941E-16,-3.));
#3574=CARTESIAN_POINT('Origin',(0.,0.,-2.));
#3575=CARTESIAN_POINT('Origin',(8.,0.,-4.));
#3576=CARTESIAN_POINT('',(-5.,6.12323399573677E-16,-4.));
#3577=CARTESIAN_POINT('Origin',(0.,0.,-4.));
#3578=CARTESIAN_POINT('Origin',(4.,0.,-2.));
#3579=CARTESIAN_POINT('',(-5.,-6.12323399573677E-16,-2.));
#3580=CARTESIAN_POINT('Origin',(0.,0.,-2.));
#3581=CARTESIAN_POINT('Origin',(0.,0.,-5.));
#3582=CARTESIAN_POINT('',(-5.,6.12323399573677E-16,12.));
#3583=CARTESIAN_POINT('Origin',(0.,0.,12.));
#3584=CARTESIAN_POINT('',(-5.,-6.12323399573677E-16,-5.));
#3585=CARTESIAN_POINT('Origin',(50.,0.,16.));
#3586=CARTESIAN_POINT('',(45.,6.12323399573677E-16,20.));
#3587=CARTESIAN_POINT('Origin',(50.,0.,20.));
#3588=CARTESIAN_POINT('',(45.,6.12323399573677E-16,12.));
#3589=CARTESIAN_POINT('',(45.,6.12323399573677E-16,16.));
#3590=CARTESIAN_POINT('Origin',(50.,0.,12.));
#3591=CARTESIAN_POINT('Origin',(50.,0.,44.));
#3592=CARTESIAN_POINT('',(2.49999999999999,-4.33012701892218,44.));
#3593=CARTESIAN_POINT('',(2.5,4.33012701892219,44.));
#3594=CARTESIAN_POINT('Origin',(0.,0.,44.));
#3595=CARTESIAN_POINT('',(0.,0.,44.));
#3596=CARTESIAN_POINT('',(0.,0.,44.));
#3597=CARTESIAN_POINT('',(100.,173.205080756888,44.));
#3598=CARTESIAN_POINT('Origin',(50.,0.,32.));
#3599=CARTESIAN_POINT('',(5.99999999999999,-10.3923048454132,32.));
#3600=CARTESIAN_POINT('',(6.,10.3923048454133,32.));
#3601=CARTESIAN_POINT('Origin',(0.,0.,32.));
#3602=CARTESIAN_POINT('',(0.,0.,32.));
#3603=CARTESIAN_POINT('',(100.,173.205080756888,32.));
#3604=CARTESIAN_POINT('',(0.,0.,32.));
#3605=CARTESIAN_POINT('Origin',(0.,0.,44.));
#3606=CARTESIAN_POINT('',(20.,34.6410161513775,44.));
#3607=CARTESIAN_POINT('',(20.,34.6410161513775,32.));
#3608=CARTESIAN_POINT('',(20.,34.6410161513775,32.));
#3609=CARTESIAN_POINT('',(0.,0.,44.));
#3610=CARTESIAN_POINT('',(0.,0.,44.));
#3611=CARTESIAN_POINT('',(0.,0.,32.));
#3612=CARTESIAN_POINT('Origin',(100.,-173.205080756888,44.));
#3613=CARTESIAN_POINT('',(20.,-34.6410161513775,32.));
#3614=CARTESIAN_POINT('',(20.,-34.6410161513775,44.));
#3615=CARTESIAN_POINT('',(20.,-34.6410161513775,32.));
#3616=CARTESIAN_POINT('',(50.,-86.6025403784438,32.));
#3617=CARTESIAN_POINT('',(50.,-86.6025403784438,44.));
#3618=CARTESIAN_POINT('Origin',(0.,0.,44.));
#3619=CARTESIAN_POINT('',(-5.,-6.12323399573677E-16,44.));
#3620=CARTESIAN_POINT('Origin',(0.,0.,44.));
#3621=CARTESIAN_POINT('Origin',(0.,0.,44.));
#3622=CARTESIAN_POINT('Origin',(0.,0.,44.));
#3623=CARTESIAN_POINT('Origin',(0.,0.,32.));
#3624=CARTESIAN_POINT('Origin',(0.,0.,32.));
#3625=CARTESIAN_POINT('',(-12.,-1.46957615897682E-15,32.));
#3626=CARTESIAN_POINT('Origin',(0.,0.,32.));
#3627=CARTESIAN_POINT('Origin',(0.,0.,32.));
#3628=CARTESIAN_POINT('Origin',(0.,0.,32.));
#3629=CARTESIAN_POINT('Origin',(0.,0.,20.));
#3630=CARTESIAN_POINT('',(-12.,-1.46957615897682E-15,20.));
#3631=CARTESIAN_POINT('',(-12.,-1.46957615897682E-15,20.));
#3632=CARTESIAN_POINT('Origin',(0.,0.,20.));
#3633=CARTESIAN_POINT('Origin',(0.,0.,20.));
#3634=CARTESIAN_POINT('',(-65.,7.9602041944578E-15,20.));
#3635=CARTESIAN_POINT('Origin',(0.,0.,20.));
#3636=CARTESIAN_POINT('Origin',(0.,0.,12.));
#3637=CARTESIAN_POINT('',(-65.,7.9602041944578E-15,12.));
#3638=CARTESIAN_POINT('Origin',(0.,0.,12.));
#3639=CARTESIAN_POINT('Origin',(0.,0.,12.));
#3640=CARTESIAN_POINT('',(-65.,-7.9602041944578E-15,12.));
#3641=CARTESIAN_POINT('Origin',(0.,0.,-5.));
#3642=CARTESIAN_POINT('',(-5.,-6.12323399573677E-16,-5.));
#3643=CARTESIAN_POINT('',(-5.,-6.12323399573677E-16,-5.));
#3644=CARTESIAN_POINT('Origin',(0.,0.,-5.));
#3645=CARTESIAN_POINT('Origin',(0.,0.,-5.));
#3646=CARTESIAN_POINT('',(-5.,-6.12323399573677E-16,60.));
#3647=CARTESIAN_POINT('Origin',(0.,0.,60.));
#3648=CARTESIAN_POINT('',(-5.,-6.12323399573677E-16,-5.));
#3649=CARTESIAN_POINT('Origin',(0.,0.,60.));
#3650=CARTESIAN_POINT('Origin',(0.,0.,-5.));
#4126=UNCERTAINTY_MEASURE_WITH_UNIT(LENGTH_MEASURE(0.01),#4150,
'DISTANCE_ACCURACY_VALUE',
'Maximum model space distance between geometric entities at asserted c
onnectivities');
#4136=UNCERTAINTY_MEASURE_WITH_UNIT(LENGTH_MEASURE(0.01),#4150,
'DISTANCE_ACCURACY_VALUE',
'Maximum model space distance between geometric entities at asserted c
onnectivities');
#4139=(
GEOMETRIC_REPRESENTATION_CONTEXT(3)
GLOBAL_UNCERTAINTY_ASSIGNED_CONTEXT((#4126))
GLOBAL_UNIT_ASSIGNED_CONTEXT((#4150,#4152,#4153))
REPRESENTATION_CONTEXT('','3D')
);
#4149=(
GEOMETRIC_REPRESENTATION_CONTEXT(3)
GLOBAL_UNCERTAINTY_ASSIGNED_CONTEXT((#4136))
GLOBAL_UNIT_ASSIGNED_CONTEXT((#4150,#4152,#4153))
REPRESENTATION_CONTEXT('','3D')
);
#4150=(
LENGTH_UNIT()
NAMED_UNIT(*)
SI_UNIT(.MILLI.,.METRE.)
);
#4152=(
NAMED_UNIT(*)
PLANE_ANGLE_UNIT()
SI_UNIT($,.RADIAN.)
);
#4153=(
NAMED_UNIT(*)
SI_UNIT($,.STERADIAN.)
SOLID_ANGLE_UNIT()
);
#4156=SHAPE_DEFINITION_REPRESENTATION(#4168,#4197);
#4168=PRODUCT_DEFINITION_SHAPE('',$,#4210);
#4197=SHAPE_REPRESENTATION('',(#2454),#4139);
#4207=PRODUCT_DEFINITION_CONTEXT('part definition',#4245,'design');
#4210=PRODUCT_DEFINITION('Driving rotor','Driving rotor',#4222,#4207);
#4222=PRODUCT_DEFINITION_FORMATION('',$,#4249);
#4245=APPLICATION_CONTEXT(
'Core Data for Automotive Mechanical Design Process');
#4246=PRODUCT_CONTEXT('part definition',#4245,'mechanical');
#4249=PRODUCT('Driving rotor','Driving rotor',$,(#4246));
#4261=PRESENTATION_STYLE_ASSIGNMENT((#4271));
#4271=SURFACE_STYLE_USAGE(.BOTH.,#4281);
#4281=SURFACE_SIDE_STYLE('',(#4291));
#4291=SURFACE_STYLE_FILL_AREA(#4301);
#4301=FILL_AREA_STYLE('Dark blue',(#4311));
#4311=FILL_AREA_STYLE_COLOUR('Dark blue',#4321);
#4321=COLOUR_RGB('Dark blue',0.0901960784313725,0.270588235294118,0.513725490196078);
ENDSEC;
END-ISO-10303-21;
